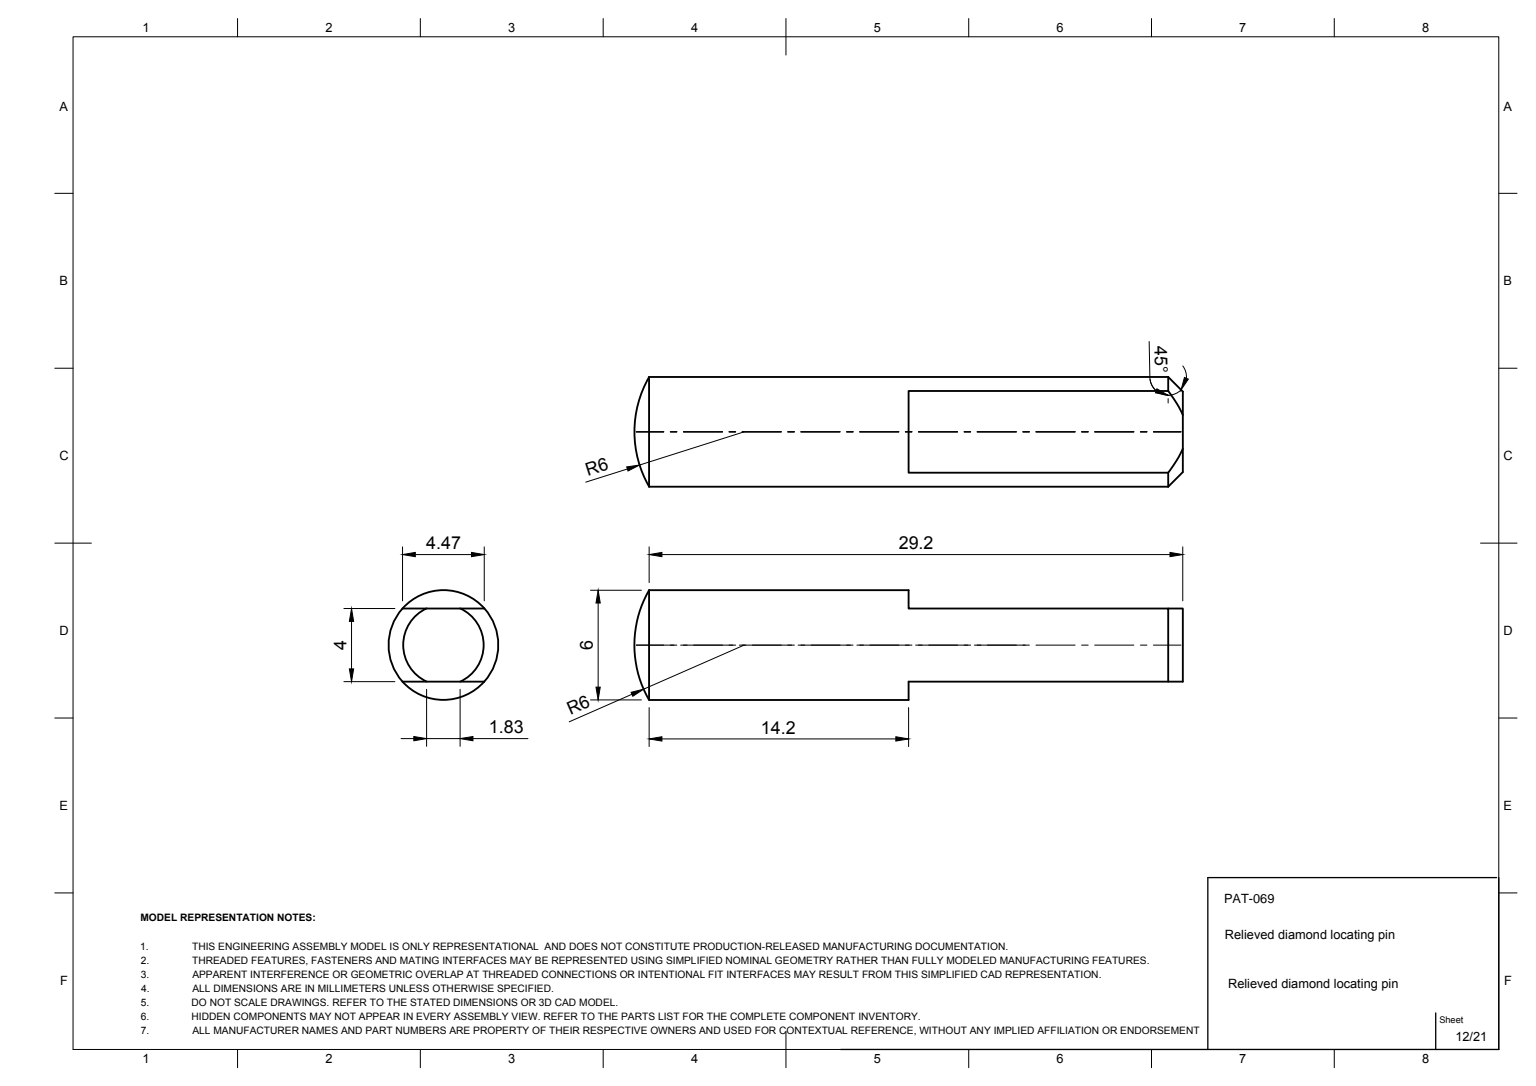
ISO-10303-21;
HEADER;
/* Generated by software containing ST-Developer
 * from STEP Tools, Inc. (www.steptools.com) 
 */

FILE_DESCRIPTION(
/* description */ ('Located fixture plate with toggle clamp'),
/* implementation_level */ '2;1');

FILE_NAME(
/* name */ 'Relieved diamond locating pin.step',
/* time_stamp */ '2026-10-27T21:36:12-07:00',
/* author */ (''),
/* organization */ (''),
/* preprocessor_version */ 'ST-DEVELOPER v20.2',
/* originating_system */ 'Autodesk Translation Framework v15.17.0.0',
/* authorisation */ '');

FILE_SCHEMA (('AUTOMOTIVE_DESIGN { 1 0 10303 214 3 1 1 }'));
ENDSEC;

DATA;
#10=MECHANICAL_DESIGN_GEOMETRIC_PRESENTATION_REPRESENTATION('',(#331),#9285);
#203=SPHERICAL_SURFACE('',#5752,0.600000000000005);
#222=(
BOUNDED_CURVE()
B_SPLINE_CURVE(2,(#8377,#8378,#8379),.UNSPECIFIED.,.F.,.F.)
B_SPLINE_CURVE_WITH_KNOTS((3,3),(0.,0.154589948065443),.UNSPECIFIED.)
CURVE()
GEOMETRIC_REPRESENTATION_ITEM()
RATIONAL_B_SPLINE_CURVE((1.,1.03384052486396,1.))
REPRESENTATION_ITEM('')
);
#223=(
BOUNDED_CURVE()
B_SPLINE_CURVE(2,(#8383,#8384,#8385),.UNSPECIFIED.,.F.,.F.)
B_SPLINE_CURVE_WITH_KNOTS((3,3),(0.,0.154589948065443),.UNSPECIFIED.)
CURVE()
GEOMETRIC_REPRESENTATION_ITEM()
RATIONAL_B_SPLINE_CURVE((1.,1.03384052486396,1.))
REPRESENTATION_ITEM('')
);
#224=(
BOUNDED_CURVE()
B_SPLINE_CURVE(2,(#8405,#8406,#8407),.UNSPECIFIED.,.F.,.F.)
B_SPLINE_CURVE_WITH_KNOTS((3,3),(0.,0.154589948065443),.UNSPECIFIED.)
CURVE()
GEOMETRIC_REPRESENTATION_ITEM()
RATIONAL_B_SPLINE_CURVE((1.,1.03384052486396,1.))
REPRESENTATION_ITEM('')
);
#225=(
BOUNDED_CURVE()
B_SPLINE_CURVE(2,(#8412,#8413,#8414),.UNSPECIFIED.,.F.,.F.)
B_SPLINE_CURVE_WITH_KNOTS((3,3),(0.,0.154589948065443),.UNSPECIFIED.)
CURVE()
GEOMETRIC_REPRESENTATION_ITEM()
RATIONAL_B_SPLINE_CURVE((1.,1.03384052486396,1.))
REPRESENTATION_ITEM('')
);
#259=CONICAL_SURFACE('',#5746,0.26,0.785398163397448);
#260=CONICAL_SURFACE('',#5753,0.26,0.785398163397448);
#283=SHAPE_REPRESENTATION_RELATIONSHIP('SRR','None',#9406,#307);
#307=ADVANCED_BREP_SHAPE_REPRESENTATION('',(#354),#9268);
#331=STYLED_ITEM('',(#9612),#354);
#354=MANIFOLD_SOLID_BREP('Body1',#5180);
#578=PLANE('',#5737);
#579=PLANE('',#5739);
#580=PLANE('',#5748);
#581=PLANE('',#5749);
#582=PLANE('',#5750);
#825=FACE_OUTER_BOUND('',#1206,.T.);
#826=FACE_OUTER_BOUND('',#1207,.T.);
#827=FACE_OUTER_BOUND('',#1208,.T.);
#828=FACE_OUTER_BOUND('',#1209,.T.);
#829=FACE_OUTER_BOUND('',#1210,.T.);
#830=FACE_OUTER_BOUND('',#1211,.T.);
#831=FACE_OUTER_BOUND('',#1212,.T.);
#832=FACE_OUTER_BOUND('',#1213,.T.);
#833=FACE_OUTER_BOUND('',#1214,.T.);
#1206=EDGE_LOOP('',(#4198,#4199));
#1207=EDGE_LOOP('',(#4200,#4201,#4202,#4203,#4204,#4205));
#1208=EDGE_LOOP('',(#4206,#4207,#4208,#4209,#4210,#4211,#4212,#4213,#4214,
#4215,#4216,#4217));
#1209=EDGE_LOOP('',(#4218,#4219,#4220,#4221));
#1210=EDGE_LOOP('',(#4222,#4223,#4224,#4225,#4226,#4227));
#1211=EDGE_LOOP('',(#4228,#4229,#4230));
#1212=EDGE_LOOP('',(#4231,#4232,#4233,#4234));
#1213=EDGE_LOOP('',(#4235));
#1214=EDGE_LOOP('',(#4236,#4237,#4238,#4239));
#1494=CIRCLE('',#5738,0.3);
#1495=CIRCLE('',#5741,0.3);
#1496=CIRCLE('',#5742,0.3);
#1497=CIRCLE('',#5743,0.3);
#1498=CIRCLE('',#5744,0.3);
#1499=CIRCLE('',#5745,0.3);
#1500=CIRCLE('',#5747,0.22);
#1501=CIRCLE('',#5751,0.22);
#1809=LINE('',#8372,#2219);
#1810=LINE('',#8375,#2220);
#1811=LINE('',#8381,#2221);
#1812=LINE('',#8386,#2222);
#1813=LINE('',#8391,#2223);
#1814=LINE('',#8395,#2224);
#1815=LINE('',#8400,#2225);
#1816=LINE('',#8409,#2226);
#1817=LINE('',#8411,#2227);
#2219=VECTOR('',#6813,1.);
#2220=VECTOR('',#6816,1.);
#2221=VECTOR('',#6817,1.);
#2222=VECTOR('',#6818,1.);
#2223=VECTOR('',#6823,1.);
#2224=VECTOR('',#6826,0.3);
#2225=VECTOR('',#6831,1.);
#2226=VECTOR('',#6840,1.);
#2227=VECTOR('',#6841,1.);
#2636=VERTEX_POINT('',#8369);
#2637=VERTEX_POINT('',#8370);
#2638=VERTEX_POINT('',#8374);
#2639=VERTEX_POINT('',#8376);
#2640=VERTEX_POINT('',#8380);
#2641=VERTEX_POINT('',#8382);
#2642=VERTEX_POINT('',#8388);
#2643=VERTEX_POINT('',#8390);
#2644=VERTEX_POINT('',#8392);
#2645=VERTEX_POINT('',#8394);
#2646=VERTEX_POINT('',#8397);
#2647=VERTEX_POINT('',#8399);
#2648=VERTEX_POINT('',#8403);
#2649=VERTEX_POINT('',#8410);
#3187=EDGE_CURVE('',#2636,#2637,#1494,.T.);
#3188=EDGE_CURVE('',#2637,#2636,#1809,.T.);
#3189=EDGE_CURVE('',#2638,#2636,#1810,.T.);
#3190=EDGE_CURVE('',#2639,#2638,#222,.T.);
#3191=EDGE_CURVE('',#2640,#2639,#1811,.T.);
#3192=EDGE_CURVE('',#2641,#2640,#223,.T.);
#3193=EDGE_CURVE('',#2637,#2641,#1812,.T.);
#3194=EDGE_CURVE('',#2642,#2641,#1495,.T.);
#3195=EDGE_CURVE('',#2642,#2643,#1813,.T.);
#3196=EDGE_CURVE('',#2643,#2644,#1496,.T.);
#3197=EDGE_CURVE('',#2644,#2645,#1814,.T.);
#3198=EDGE_CURVE('',#2645,#2645,#1497,.T.);
#3199=EDGE_CURVE('',#2644,#2646,#1498,.T.);
#3200=EDGE_CURVE('',#2646,#2647,#1815,.T.);
#3201=EDGE_CURVE('',#2638,#2647,#1499,.T.);
#3202=EDGE_CURVE('',#2648,#2640,#1500,.T.);
#3203=EDGE_CURVE('',#2648,#2642,#224,.T.);
#3204=EDGE_CURVE('',#2643,#2646,#1816,.T.);
#3205=EDGE_CURVE('',#2649,#2648,#1817,.T.);
#3206=EDGE_CURVE('',#2647,#2649,#225,.T.);
#3207=EDGE_CURVE('',#2639,#2649,#1501,.T.);
#4198=ORIENTED_EDGE('',*,*,#3187,.F.);
#4199=ORIENTED_EDGE('',*,*,#3188,.F.);
#4200=ORIENTED_EDGE('',*,*,#3189,.F.);
#4201=ORIENTED_EDGE('',*,*,#3190,.F.);
#4202=ORIENTED_EDGE('',*,*,#3191,.F.);
#4203=ORIENTED_EDGE('',*,*,#3192,.F.);
#4204=ORIENTED_EDGE('',*,*,#3193,.F.);
#4205=ORIENTED_EDGE('',*,*,#3188,.T.);
#4206=ORIENTED_EDGE('',*,*,#3189,.T.);
#4207=ORIENTED_EDGE('',*,*,#3187,.T.);
#4208=ORIENTED_EDGE('',*,*,#3193,.T.);
#4209=ORIENTED_EDGE('',*,*,#3194,.F.);
#4210=ORIENTED_EDGE('',*,*,#3195,.T.);
#4211=ORIENTED_EDGE('',*,*,#3196,.T.);
#4212=ORIENTED_EDGE('',*,*,#3197,.T.);
#4213=ORIENTED_EDGE('',*,*,#3198,.T.);
#4214=ORIENTED_EDGE('',*,*,#3197,.F.);
#4215=ORIENTED_EDGE('',*,*,#3199,.T.);
#4216=ORIENTED_EDGE('',*,*,#3200,.T.);
#4217=ORIENTED_EDGE('',*,*,#3201,.F.);
#4218=ORIENTED_EDGE('',*,*,#3192,.T.);
#4219=ORIENTED_EDGE('',*,*,#3202,.F.);
#4220=ORIENTED_EDGE('',*,*,#3203,.T.);
#4221=ORIENTED_EDGE('',*,*,#3194,.T.);
#4222=ORIENTED_EDGE('',*,*,#3200,.F.);
#4223=ORIENTED_EDGE('',*,*,#3204,.F.);
#4224=ORIENTED_EDGE('',*,*,#3195,.F.);
#4225=ORIENTED_EDGE('',*,*,#3203,.F.);
#4226=ORIENTED_EDGE('',*,*,#3205,.F.);
#4227=ORIENTED_EDGE('',*,*,#3206,.F.);
#4228=ORIENTED_EDGE('',*,*,#3196,.F.);
#4229=ORIENTED_EDGE('',*,*,#3204,.T.);
#4230=ORIENTED_EDGE('',*,*,#3199,.F.);
#4231=ORIENTED_EDGE('',*,*,#3191,.T.);
#4232=ORIENTED_EDGE('',*,*,#3207,.T.);
#4233=ORIENTED_EDGE('',*,*,#3205,.T.);
#4234=ORIENTED_EDGE('',*,*,#3202,.T.);
#4235=ORIENTED_EDGE('',*,*,#3198,.F.);
#4236=ORIENTED_EDGE('',*,*,#3190,.T.);
#4237=ORIENTED_EDGE('',*,*,#3201,.T.);
#4238=ORIENTED_EDGE('',*,*,#3206,.T.);
#4239=ORIENTED_EDGE('',*,*,#3207,.F.);
#4842=CYLINDRICAL_SURFACE('',#5740,0.3);
#5026=ADVANCED_FACE('',(#825),#578,.F.);
#5027=ADVANCED_FACE('',(#826),#579,.T.);
#5028=ADVANCED_FACE('',(#827),#4842,.T.);
#5029=ADVANCED_FACE('',(#828),#259,.T.);
#5030=ADVANCED_FACE('',(#829),#580,.F.);
#5031=ADVANCED_FACE('',(#830),#581,.F.);
#5032=ADVANCED_FACE('',(#831),#582,.T.);
#5033=ADVANCED_FACE('',(#832),#203,.T.);
#5034=ADVANCED_FACE('',(#833),#260,.T.);
#5180=CLOSED_SHELL('',(#5026,#5027,#5028,#5029,#5030,#5031,#5032,#5033,
#5034));
#5736=AXIS2_PLACEMENT_3D('',#8367,#6807,#6808);
#5737=AXIS2_PLACEMENT_3D('',#8368,#6809,#6810);
#5738=AXIS2_PLACEMENT_3D('',#8371,#6811,#6812);
#5739=AXIS2_PLACEMENT_3D('',#8373,#6814,#6815);
#5740=AXIS2_PLACEMENT_3D('',#8387,#6819,#6820);
#5741=AXIS2_PLACEMENT_3D('',#8389,#6821,#6822);
#5742=AXIS2_PLACEMENT_3D('',#8393,#6824,#6825);
#5743=AXIS2_PLACEMENT_3D('',#8396,#6827,#6828);
#5744=AXIS2_PLACEMENT_3D('',#8398,#6829,#6830);
#5745=AXIS2_PLACEMENT_3D('',#8401,#6832,#6833);
#5746=AXIS2_PLACEMENT_3D('',#8402,#6834,#6835);
#5747=AXIS2_PLACEMENT_3D('',#8404,#6836,#6837);
#5748=AXIS2_PLACEMENT_3D('',#8408,#6838,#6839);
#5749=AXIS2_PLACEMENT_3D('',#8415,#6842,#6843);
#5750=AXIS2_PLACEMENT_3D('',#8416,#6844,#6845);
#5751=AXIS2_PLACEMENT_3D('',#8417,#6846,#6847);
#5752=AXIS2_PLACEMENT_3D('',#8418,#6848,#6849);
#5753=AXIS2_PLACEMENT_3D('',#8419,#6850,#6851);
#6807=DIRECTION('axis',(0.,0.,1.));
#6808=DIRECTION('refdir',(1.,0.,0.));
#6809=DIRECTION('center_axis',(0.,1.,0.));
#6810=DIRECTION('ref_axis',(0.,0.,1.));
#6811=DIRECTION('center_axis',(0.,1.,0.));
#6812=DIRECTION('ref_axis',(1.,0.,0.));
#6813=DIRECTION('',(0.,0.,1.));
#6814=DIRECTION('center_axis',(1.,0.,0.));
#6815=DIRECTION('ref_axis',(0.,0.,-1.));
#6816=DIRECTION('',(0.,1.,0.));
#6817=DIRECTION('',(0.,0.,1.));
#6818=DIRECTION('',(0.,-1.,0.));
#6819=DIRECTION('center_axis',(0.,-1.,0.));
#6820=DIRECTION('ref_axis',(1.,0.,0.));
#6821=DIRECTION('center_axis',(0.,-1.,0.));
#6822=DIRECTION('ref_axis',(1.,0.,0.));
#6823=DIRECTION('',(0.,1.,0.));
#6824=DIRECTION('center_axis',(0.,1.,0.));
#6825=DIRECTION('ref_axis',(1.,0.,0.));
#6826=DIRECTION('',(0.,1.,0.));
#6827=DIRECTION('center_axis',(0.,-1.,0.));
#6828=DIRECTION('ref_axis',(1.,0.,0.));
#6829=DIRECTION('center_axis',(0.,1.,0.));
#6830=DIRECTION('ref_axis',(1.,0.,0.));
#6831=DIRECTION('',(0.,-1.,0.));
#6832=DIRECTION('center_axis',(0.,-1.,0.));
#6833=DIRECTION('ref_axis',(1.,0.,0.));
#6834=DIRECTION('center_axis',(0.,1.,0.));
#6835=DIRECTION('ref_axis',(1.,0.,0.));
#6836=DIRECTION('center_axis',(0.,-1.,0.));
#6837=DIRECTION('ref_axis',(1.,0.,0.));
#6838=DIRECTION('center_axis',(1.,0.,0.));
#6839=DIRECTION('ref_axis',(0.,0.,-1.));
#6840=DIRECTION('',(0.,0.,1.));
#6841=DIRECTION('',(0.,0.,-1.));
#6842=DIRECTION('center_axis',(0.,1.,0.));
#6843=DIRECTION('ref_axis',(0.,0.,1.));
#6844=DIRECTION('center_axis',(0.,-1.,0.));
#6845=DIRECTION('ref_axis',(0.,0.,-1.));
#6846=DIRECTION('center_axis',(0.,-1.,0.));
#6847=DIRECTION('ref_axis',(1.,0.,0.));
#6848=DIRECTION('center_axis',(6.12323399573677E-17,0.,1.));
#6849=DIRECTION('ref_axis',(1.,0.,0.));
#6850=DIRECTION('center_axis',(0.,1.,0.));
#6851=DIRECTION('ref_axis',(1.,0.,0.));
#8367=CARTESIAN_POINT('',(0.,0.,0.));
#8368=CARTESIAN_POINT('Origin',(0.2,1.5,-0.4));
#8369=CARTESIAN_POINT('',(0.2,1.5,0.223606797749979));
#8370=CARTESIAN_POINT('',(0.2,1.5,-0.223606797749979));
#8371=CARTESIAN_POINT('Origin',(0.,1.5,0.));
#8372=CARTESIAN_POINT('',(0.2,1.5,-0.4));
#8373=CARTESIAN_POINT('Origin',(0.2,0.7,0.));
#8374=CARTESIAN_POINT('',(0.2,0.08,0.223606797749979));
#8375=CARTESIAN_POINT('',(0.2,1.49980762113533,0.223606797749979));
#8376=CARTESIAN_POINT('',(0.2,0.,0.0916515138991168));
#8377=CARTESIAN_POINT('Ctrl Pts',(0.2,0.,0.0916515138991168));
#8378=CARTESIAN_POINT('Ctrl Pts',(0.2,0.0232575029459984,0.147478749374482));
#8379=CARTESIAN_POINT('Ctrl Pts',(0.2,0.08,0.223606797749979));
#8380=CARTESIAN_POINT('',(0.2,0.,-0.0916515138991168));
#8381=CARTESIAN_POINT('',(0.2,0.,0.));
#8382=CARTESIAN_POINT('',(0.2,0.08,-0.223606797749979));
#8383=CARTESIAN_POINT('Ctrl Pts',(0.2,0.08,-0.223606797749979));
#8384=CARTESIAN_POINT('Ctrl Pts',(0.2,0.0232575029459984,-0.147478749374482));
#8385=CARTESIAN_POINT('Ctrl Pts',(0.2,0.,-0.0916515138991168));
#8386=CARTESIAN_POINT('',(0.2,1.49980762113533,-0.223606797749979));
#8387=CARTESIAN_POINT('Origin',(0.,1.49980762113533,0.));
#8388=CARTESIAN_POINT('',(-0.2,0.08,-0.223606797749979));
#8389=CARTESIAN_POINT('Origin',(0.,0.08,0.));
#8390=CARTESIAN_POINT('',(-0.2,1.5,-0.223606797749979));
#8391=CARTESIAN_POINT('',(-0.2,1.49980762113533,-0.223606797749979));
#8392=CARTESIAN_POINT('',(-0.3,1.5,-3.67394039744206E-17));
#8393=CARTESIAN_POINT('Origin',(0.,1.5,0.));
#8394=CARTESIAN_POINT('',(-0.3,2.91961524227066,-3.67394039744206E-17));
#8395=CARTESIAN_POINT('',(-0.3,1.49980762113533,-3.67394039744206E-17));
#8396=CARTESIAN_POINT('Origin',(0.,2.91961524227066,0.));
#8397=CARTESIAN_POINT('',(-0.2,1.5,0.223606797749979));
#8398=CARTESIAN_POINT('Origin',(0.,1.5,0.));
#8399=CARTESIAN_POINT('',(-0.2,0.08,0.223606797749979));
#8400=CARTESIAN_POINT('',(-0.2,1.49980762113533,0.223606797749979));
#8401=CARTESIAN_POINT('Origin',(0.,0.08,0.));
#8402=CARTESIAN_POINT('Origin',(0.,0.04,0.));
#8403=CARTESIAN_POINT('',(-0.2,0.,-0.0916515138991168));
#8404=CARTESIAN_POINT('Origin',(0.,0.,0.));
#8405=CARTESIAN_POINT('Ctrl Pts',(-0.2,0.,-0.0916515138991168));
#8406=CARTESIAN_POINT('Ctrl Pts',(-0.2,0.0232575029459984,-0.147478749374482));
#8407=CARTESIAN_POINT('Ctrl Pts',(-0.2,0.08,-0.223606797749979));
#8408=CARTESIAN_POINT('Origin',(-0.2,0.7,0.));
#8409=CARTESIAN_POINT('',(-0.2,1.5,-0.4));
#8410=CARTESIAN_POINT('',(-0.2,0.,0.0916515138991168));
#8411=CARTESIAN_POINT('',(-0.2,0.,0.));
#8412=CARTESIAN_POINT('Ctrl Pts',(-0.2,0.08,0.223606797749979));
#8413=CARTESIAN_POINT('Ctrl Pts',(-0.2,0.0232575029459984,0.147478749374482));
#8414=CARTESIAN_POINT('Ctrl Pts',(-0.2,0.,0.0916515138991168));
#8415=CARTESIAN_POINT('Origin',(-0.4,1.5,-0.4));
#8416=CARTESIAN_POINT('Origin',(0.,0.,0.));
#8417=CARTESIAN_POINT('Origin',(0.,0.,0.));
#8418=CARTESIAN_POINT('Origin',(-8.04911692853238E-16,2.4,0.));
#8419=CARTESIAN_POINT('Origin',(0.,0.04,0.));
#9238=UNCERTAINTY_MEASURE_WITH_UNIT(LENGTH_MEASURE(0.001),#9286,
'DISTANCE_ACCURACY_VALUE',
'Maximum model space distance between geometric entities at asserted c
onnectivities');
#9255=UNCERTAINTY_MEASURE_WITH_UNIT(LENGTH_MEASURE(0.001),#9286,
'DISTANCE_ACCURACY_VALUE',
'Maximum model space distance between geometric entities at asserted c
onnectivities');
#9268=(
GEOMETRIC_REPRESENTATION_CONTEXT(3)
GLOBAL_UNCERTAINTY_ASSIGNED_CONTEXT((#9238))
GLOBAL_UNIT_ASSIGNED_CONTEXT((#9286,#9288,#9289))
REPRESENTATION_CONTEXT('','3D')
);
#9285=(
GEOMETRIC_REPRESENTATION_CONTEXT(3)
GLOBAL_UNCERTAINTY_ASSIGNED_CONTEXT((#9255))
GLOBAL_UNIT_ASSIGNED_CONTEXT((#9286,#9288,#9289))
REPRESENTATION_CONTEXT('','3D')
);
#9286=(
LENGTH_UNIT()
NAMED_UNIT(*)
SI_UNIT(.CENTI.,.METRE.)
);
#9288=(
NAMED_UNIT(*)
PLANE_ANGLE_UNIT()
SI_UNIT($,.RADIAN.)
);
#9289=(
NAMED_UNIT(*)
SI_UNIT($,.STERADIAN.)
SOLID_ANGLE_UNIT()
);
#9302=SHAPE_DEFINITION_REPRESENTATION(#9331,#9406);
#9331=PRODUCT_DEFINITION_SHAPE('',$,#9436);
#9406=SHAPE_REPRESENTATION('',(#5736),#9268);
#9423=PRODUCT_DEFINITION_CONTEXT('part definition',#9512,'design');
#9436=PRODUCT_DEFINITION('Relieved diamond locating pin',
'Relieved diamond locating pin',#9465,#9423);
#9465=PRODUCT_DEFINITION_FORMATION('',$,#9526);
#9512=APPLICATION_CONTEXT(
'Core Data for Automotive Mechanical Design Process');
#9513=PRODUCT_CONTEXT('part definition',#9512,'mechanical');
#9526=PRODUCT('Relieved diamond locating pin',
'Relieved diamond locating pin','Relieved diamond locating pin',(#9513));
#9606=COLOUR_RGB('Grey',0.48,0.52,0.57);
#9607=FILL_AREA_STYLE_COLOUR('',#9606);
#9608=FILL_AREA_STYLE('',(#9607));
#9609=SURFACE_STYLE_FILL_AREA(#9608);
#9610=SURFACE_SIDE_STYLE('',(#9609));
#9611=SURFACE_STYLE_USAGE(.BOTH.,#9610);
#9612=PRESENTATION_STYLE_ASSIGNMENT((#9611));
ENDSEC;
END-ISO-10303-21;
